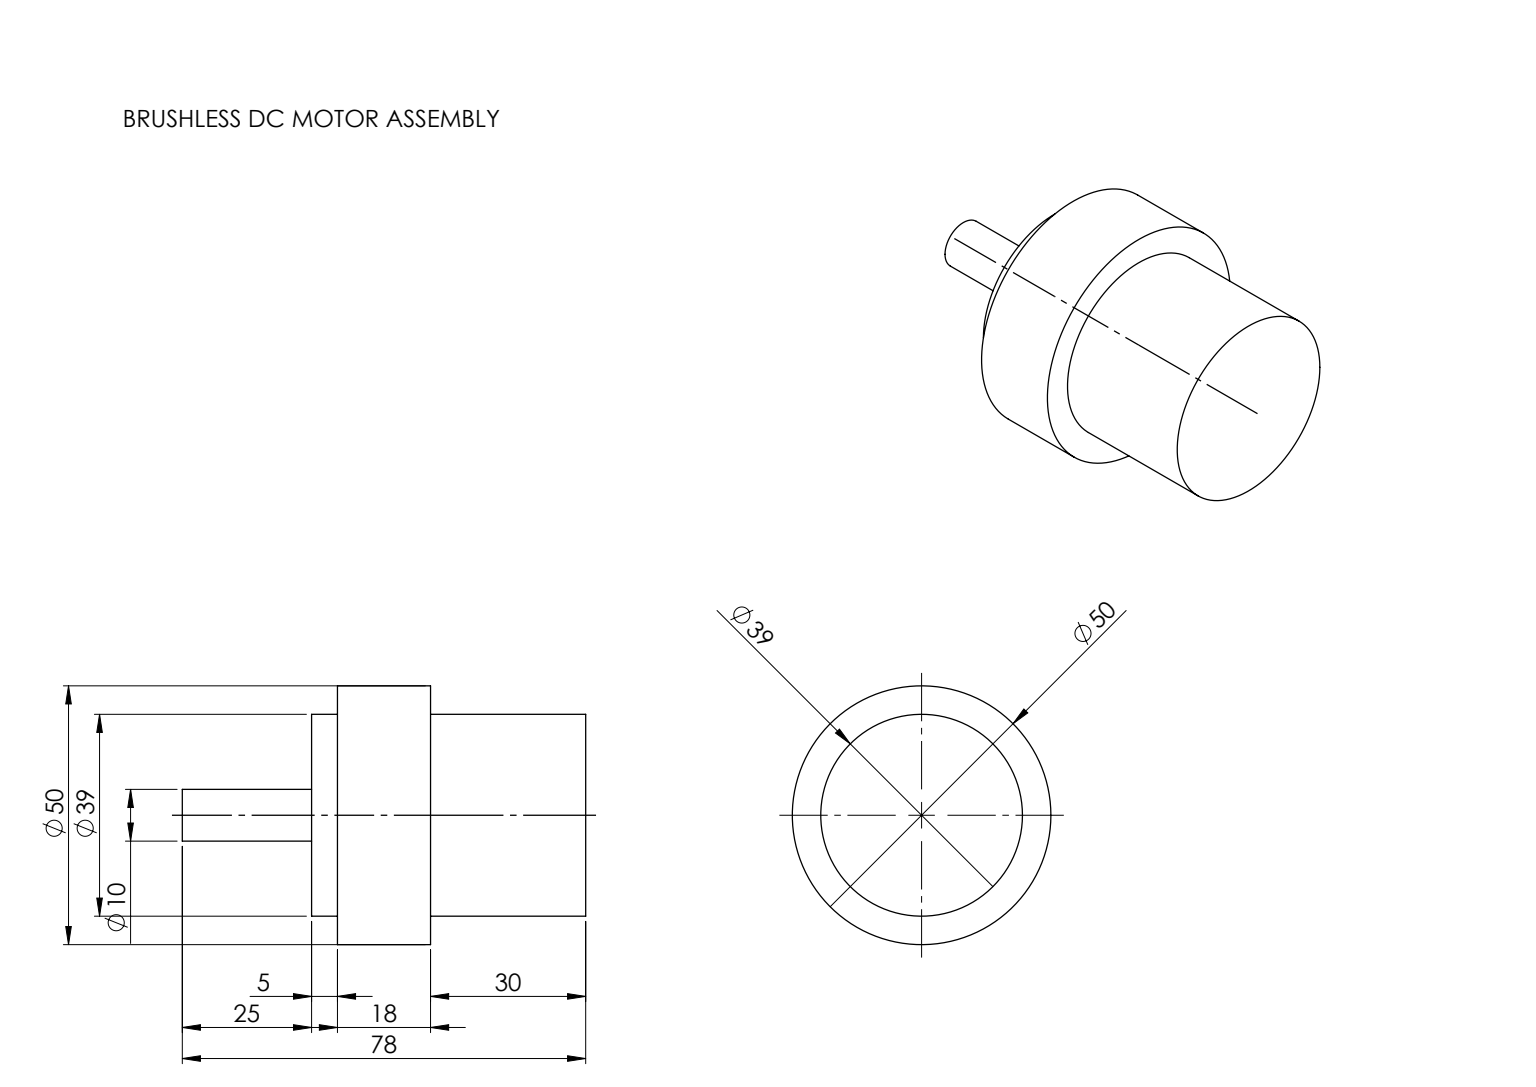
ISO-10303-21;
HEADER;
FILE_DESCRIPTION (('STEP AP214'),
    '1' );
FILE_NAME ('Brushless DC Motor Assembly.step',
    '2026-10-05T20:22:16',
    ( '' ),
    ( '' ),
    'SwSTEP 2.0',
    'SolidWorks 2026',
    '' );
FILE_SCHEMA (( 'AUTOMOTIVE_DESIGN' ));
ENDSEC;

DATA;
#83=ORIENTED_EDGE ( 'NONE', *, *, #15385, .F. ) ;
#148=( LENGTH_UNIT ( ) NAMED_UNIT ( * ) SI_UNIT ( .MILLI., .METRE. ) );
#153=CYLINDRICAL_SURFACE ( 'NONE', #9538, 24.99999999999999645 ) ;
#181=CARTESIAN_POINT ( 'NONE',  ( -50.00000000000000000, 171.6227766016838245, 0.000000000000000000 ) ) ;
#284=CARTESIAN_POINT ( 'NONE',  ( -68.00000000000000000, 171.6227766016838245, 24.99999999999999289 ) ) ;
#327=PRESENTATION_STYLE_ASSIGNMENT (( #16528 ) ) ;
#375=CARTESIAN_POINT ( 'NONE',  ( -68.00000000000000000, 171.6227766016838245, -19.49999999999999645 ) ) ;
#389=EDGE_LOOP ( 'NONE', ( #662, #9822, #5339, #17357 ) ) ;
#493=ORIENTED_EDGE ( 'NONE', *, *, #9337, .F. ) ;
#506=VECTOR ( 'NONE', #763, 1000.000000000000000 ) ;
#507=ORIENTED_EDGE ( 'NONE', *, *, #5137, .F. ) ;
#527=DIRECTION ( 'NONE',  ( 1.000000000000000000, -0.000000000000000000, -0.000000000000000000 ) ) ;
#616=DIRECTION ( 'NONE',  ( 0.000000000000000000, 0.000000000000000000, 1.000000000000000000 ) ) ;
#628=EDGE_CURVE ( 'NONE', #9656, #12025, #15580, .T. ) ;
#636=CARTESIAN_POINT ( 'NONE',  ( -68.00000000000000000, 171.6227766016838245, 0.000000000000000000 ) ) ;
#662=ORIENTED_EDGE ( 'NONE', *, *, #10245, .F. ) ;
#746=DIRECTION ( 'NONE',  ( 0.000000000000000000, 0.000000000000000000, 1.000000000000000000 ) ) ;
#751=DIRECTION ( 'NONE',  ( -1.000000000000000000, 0.000000000000000000, 0.000000000000000000 ) ) ;
#763=DIRECTION ( 'NONE',  ( -1.000000000000000000, -0.000000000000000000, -0.000000000000000000 ) ) ;
#908=ORIENTED_EDGE ( 'NONE', *, *, #8104, .T. ) ;
#928=ORIENTED_EDGE ( 'NONE', *, *, #4621, .F. ) ;
#989=FACE_OUTER_BOUND ( 'NONE', #6924, .T. ) ;
#992=DIRECTION ( 'NONE',  ( -1.000000000000000000, 0.000000000000000000, 0.000000000000000000 ) ) ;
#1039=AXIS2_PLACEMENT_3D ( 'NONE', #16734, #11404, #12560 ) ;
#1159=ADVANCED_FACE ( 'NONE', ( #4225 ), #17507, .T. ) ;
#1236=DIRECTION ( 'NONE',  ( 1.000000000000000000, 0.000000000000000000, -0.000000000000000000 ) ) ;
#1281=DIRECTION ( 'NONE',  ( 0.000000000000000000, 0.000000000000000000, 1.000000000000000000 ) ) ;
#1300=AXIS2_PLACEMENT_3D ( 'NONE', #2966, #10847, #2802 ) ;
#1345=COLOUR_RGB ( '', 0.08235294, 0.09019608, 0.10196078) ;
#1351=PRODUCT_DEFINITION ( 'UNKNOWN', '', #8975, #12448 ) ;
#1374=ORIENTED_EDGE ( 'NONE', *, *, #14927, .T. ) ;
#1493=PLANE ( 'NONE',  #4122 ) ;
#1524=DIRECTION ( 'NONE',  ( 1.000000000000000000, 0.000000000000000000, 0.000000000000000000 ) ) ;
#1543=CARTESIAN_POINT ( 'NONE',  ( -73.00000000000001421, 171.6227766016838245, 5.000000000000006217 ) ) ;
#1546=FACE_OUTER_BOUND ( 'NONE', #389, .T. ) ;
#1562=SURFACE_SIDE_STYLE ('',( #10778 ) ) ;
#1574=EDGE_CURVE ( 'NONE', #14903, #9038, #2433, .T. ) ;
#1722=AXIS2_PLACEMENT_3D ( 'NONE', #2794, #16251, #2704 ) ;
#1774=ORIENTED_EDGE ( 'NONE', *, *, #8939, .F. ) ;
#1789=CARTESIAN_POINT ( 'NONE',  ( -68.00000000000000000, 171.6227766016838245, -25.00000000000000000 ) ) ;
#1833=PLANE ( 'NONE',  #14966 ) ;
#1897=CARTESIAN_POINT ( 'NONE',  ( -50.00000000000000000, 171.6227766016838245, -2.296212748401287183E-15 ) ) ;
#1995=CARTESIAN_POINT ( 'NONE',  ( -20.00000000000000355, 171.6227766016838245, 19.49999999999998934 ) ) ;
#2011=AXIS2_PLACEMENT_3D ( 'NONE', #636, #9923, #3019 ) ;
#2016=CARTESIAN_POINT ( 'NONE',  ( -73.00000000000001421, 171.6227766016838245, 19.49999999999999645 ) ) ;
#2021=ADVANCED_FACE ( 'NONE', ( #14578 ), #2450, .T. ) ;
#2078=ORIENTED_EDGE ( 'NONE', *, *, #17126, .F. ) ;
#2104=ORIENTED_EDGE ( 'NONE', *, *, #6682, .T. ) ;
#2130=CARTESIAN_POINT ( 'NONE',  ( -138.7106781186547266, 171.6227766016838245, -25.00000000000000000 ) ) ;
#2157=DIRECTION ( 'NONE',  ( 0.000000000000000000, 0.000000000000000000, 1.000000000000000000 ) ) ;
#2167=ORIENTED_EDGE ( 'NONE', *, *, #4621, .T. ) ;
#2199=( LENGTH_UNIT ( ) NAMED_UNIT ( * ) SI_UNIT ( .MILLI., .METRE. ) );
#2383=DIRECTION ( 'NONE',  ( 0.000000000000000000, 0.000000000000000000, 1.000000000000000000 ) ) ;
#2387=AXIS2_PLACEMENT_3D ( 'NONE', #8252, #1524, #6920 ) ;
#2393=ORIENTED_EDGE ( 'NONE', *, *, #14927, .F. ) ;
#2433=CIRCLE ( 'NONE', #6680, 19.49999999999999645 ) ;
#2450=CYLINDRICAL_SURFACE ( 'NONE', #12720, 24.99999999999999645 ) ;
#2520=EDGE_CURVE ( 'NONE', #6066, #5020, #9110, .T. ) ;
#2642=EDGE_LOOP ( 'NONE', ( #17068, #9628, #2768, #7721 ) ) ;
#2652=ORIENTED_EDGE ( 'NONE', *, *, #10245, .T. ) ;
#2690=CARTESIAN_POINT ( 'NONE',  ( -50.00000000000000000, 171.6227766016838245, -19.49999999999998934 ) ) ;
#2704=DIRECTION ( 'NONE',  ( 0.000000000000000000, 0.000000000000000000, -1.000000000000000000 ) ) ;
#2707=CIRCLE ( 'NONE', #12597, 19.49999999999998934 ) ;
#2727=CLOSED_SHELL ( 'NONE', ( #6033, #12737, #9025, #2021, #13496, #6623, #3604, #8684, #14834, #3442, #10301, #1159, #11380 ) ) ;
#2768=ORIENTED_EDGE ( 'NONE', *, *, #7492, .T. ) ;
#2790=SHAPE_DEFINITION_REPRESENTATION ( #14917, #17442 ) ;
#2794=CARTESIAN_POINT ( 'NONE',  ( -73.00000000000001421, 171.6227766016838245, 0.000000000000000000 ) ) ;
#2802=DIRECTION ( 'NONE',  ( 0.000000000000000000, 0.000000000000000000, -1.000000000000000000 ) ) ;
#2923=DIRECTION ( 'NONE',  ( 0.000000000000000000, 0.000000000000000000, -1.000000000000000000 ) ) ;
#2936=DIRECTION ( 'NONE',  ( -1.000000000000000000, -0.000000000000000000, -0.000000000000000000 ) ) ;
#2966=CARTESIAN_POINT ( 'NONE',  ( -50.00000000000000000, 171.6227766016838245, -2.296212748401287183E-15 ) ) ;
#2969=DIRECTION ( 'NONE',  ( 0.000000000000000000, 0.000000000000000000, -1.000000000000000000 ) ) ;
#2974=( NAMED_UNIT ( * ) PLANE_ANGLE_UNIT ( ) SI_UNIT ( $, .RADIAN. ) );
#3019=DIRECTION ( 'NONE',  ( 0.000000000000000000, 0.000000000000000000, 1.000000000000000000 ) ) ;
#3082=CIRCLE ( 'NONE', #13271, 24.99999999999999645 ) ;
#3103=ORIENTED_EDGE ( 'NONE', *, *, #7492, .F. ) ;
#3189=EDGE_LOOP ( 'NONE', ( #2167, #14857 ) ) ;
#3217=VERTEX_POINT ( 'NONE', #7731 ) ;
#3225=VERTEX_POINT ( 'NONE', #7568 ) ;
#3227=DIRECTION ( 'NONE',  ( 1.000000000000000000, -0.000000000000000000, -0.000000000000000000 ) ) ;
#3256=COLOUR_RGB ( '', 0.08235294, 0.09019608, 0.10196078) ;
#3280=CARTESIAN_POINT ( 'NONE',  ( -73.00000000000001421, 171.6227766016838245, 0.000000000000000000 ) ) ;
#3308=CIRCLE ( 'NONE', #7822, 5.000000000000006217 ) ;
#3377=CIRCLE ( 'NONE', #6186, 5.000000000000006217 ) ;
#3407=CYLINDRICAL_SURFACE ( 'NONE', #14893, 19.49999999999998934 ) ;
#3431=LINE ( 'NONE', #2016, #6489 ) ;
#3442=ADVANCED_FACE ( 'NONE', ( #9595 ), #14998, .T. ) ;
#3530=VECTOR ( 'NONE', #14519, 1000.000000000000000 ) ;
#3583=AXIS2_PLACEMENT_3D ( 'NONE', #5482, #6893, #8222 ) ;
#3604=ADVANCED_FACE ( 'NONE', ( #11764, #13191 ), #4001, .F. ) ;
#3626=AXIS2_PLACEMENT_3D ( 'NONE', #13286, #1236, #2383 ) ;
#3652=ORIENTED_EDGE ( 'NONE', *, *, #5137, .T. ) ;
#3715=CIRCLE ( 'NONE', #4287, 5.000000000000006217 ) ;
#3819=DIRECTION ( 'NONE',  ( 0.000000000000000000, 0.000000000000000000, -1.000000000000000000 ) ) ;
#3834=CYLINDRICAL_SURFACE ( 'NONE', #12341, 5.000000000000006217 ) ;
#3877=EDGE_LOOP ( 'NONE', ( #4904, #2393 ) ) ;
#3989=AXIS2_PLACEMENT_3D ( 'NONE', #5717, #3227, #11105 ) ;
#4001=PLANE ( 'NONE',  #3626 ) ;
#4025=DIRECTION ( 'NONE',  ( 0.000000000000000000, 0.000000000000000000, -1.000000000000000000 ) ) ;
#4122=AXIS2_PLACEMENT_3D ( 'NONE', #9711, #9626, #4240 ) ;
#4137=FILL_AREA_STYLE_COLOUR ( '', #1345 ) ;
#4154=ORIENTED_EDGE ( 'NONE', *, *, #8876, .T. ) ;
#4159=AXIS2_PLACEMENT_3D ( 'NONE', #11837, #11661, #10329 ) ;
#4173=CIRCLE ( 'NONE', #4159, 5.000000000000006217 ) ;
#4175=DIRECTION ( 'NONE',  ( 1.000000000000000000, 0.000000000000000000, 0.000000000000000000 ) ) ;
#4225=FACE_OUTER_BOUND ( 'NONE', #9263, .T. ) ;
#4240=DIRECTION ( 'NONE',  ( 0.000000000000000000, 0.000000000000000000, 1.000000000000000000 ) ) ;
#4243=ORIENTED_EDGE ( 'NONE', *, *, #17126, .T. ) ;
#4287=AXIS2_PLACEMENT_3D ( 'NONE', #15608, #992, #9133 ) ;
#4401=( NAMED_UNIT ( * ) SI_UNIT ( $, .STERADIAN. ) SOLID_ANGLE_UNIT ( ) );
#4507=ORIENTED_EDGE ( 'NONE', *, *, #7212, .F. ) ;
#4571=PLANE ( 'NONE',  #10997 ) ;
#4621=EDGE_CURVE ( 'NONE', #5464, #5020, #3082, .T. ) ;
#4692=( NAMED_UNIT ( * ) SI_UNIT ( $, .STERADIAN. ) SOLID_ANGLE_UNIT ( ) );
#4720=VERTEX_POINT ( 'NONE', #6227 ) ;
#4750=ORIENTED_EDGE ( 'NONE', *, *, #1574, .F. ) ;
#4904=ORIENTED_EDGE ( 'NONE', *, *, #13206, .F. ) ;
#4938=DIRECTION ( 'NONE',  ( 1.000000000000000000, 0.000000000000000000, 0.000000000000000000 ) ) ;
#4992=VECTOR ( 'NONE', #8844, 1000.000000000000000 ) ;
#5020=VERTEX_POINT ( 'NONE', #12936 ) ;
#5032=SURFACE_STYLE_USAGE ( .BOTH. , #15836 ) ;
#5137=EDGE_CURVE ( 'NONE', #6998, #13633, #15759, .T. ) ;
#5139=DIRECTION ( 'NONE',  ( 1.000000000000000000, 0.000000000000000000, 0.000000000000000000 ) ) ;
#5231=DIRECTION ( 'NONE',  ( 0.000000000000000000, 0.000000000000000000, 1.000000000000000000 ) ) ;
#5271=EDGE_CURVE ( 'NONE', #3217, #5676, #17416, .T. ) ;
#5339=ORIENTED_EDGE ( 'NONE', *, *, #8939, .T. ) ;
#5378=CARTESIAN_POINT ( 'NONE',  ( -98.00000000000000000, 171.6227766016838245, 0.000000000000000000 ) ) ;
#5396=DIRECTION ( 'NONE',  ( 0.000000000000000000, 0.000000000000000000, -1.000000000000000000 ) ) ;
#5420=CARTESIAN_POINT ( 'NONE',  ( -20.00000000000000355, 171.6227766016838245, 0.000000000000000000 ) ) ;
#5464=VERTEX_POINT ( 'NONE', #15892 ) ;
#5482=CARTESIAN_POINT ( 'NONE',  ( 0.000000000000000000, 0.000000000000000000, 0.000000000000000000 ) ) ;
#5593=PRODUCT ( 'Brushless DC Motor Assembly', 'Brushless DC Motor Assembly', '', ( #12343 ) ) ;
#5676=VERTEX_POINT ( 'NONE', #1543 ) ;
#5717=CARTESIAN_POINT ( 'NONE',  ( -73.00000000000001421, 171.6227766016838245, 0.000000000000000000 ) ) ;
#6008=EDGE_LOOP ( 'NONE', ( #7802, #11194, #4243, #8727 ) ) ;
#6033=ADVANCED_FACE ( 'NONE', ( #989 ), #3834, .T. ) ;
#6066=VERTEX_POINT ( 'NONE', #284 ) ;
#6160=ORIENTED_EDGE ( 'NONE', *, *, #10501, .F. ) ;
#6185=CARTESIAN_POINT ( 'NONE',  ( -20.00000000000000355, 171.6227766016838245, 0.000000000000000000 ) ) ;
#6186=AXIS2_PLACEMENT_3D ( 'NONE', #15789, #9059, #2157 ) ;
#6227=CARTESIAN_POINT ( 'NONE',  ( -68.00000000000000000, 171.6227766016838245, 19.49999999999999645 ) ) ;
#6489=VECTOR ( 'NONE', #11648, 1000.000000000000000 ) ;
#6623=ADVANCED_FACE ( 'NONE', ( #13817, #13907 ), #7163, .T. ) ;
#6657=EDGE_CURVE ( 'NONE', #3217, #6998, #3308, .T. ) ;
#6680=AXIS2_PLACEMENT_3D ( 'NONE', #3280, #8686, #14092 ) ;
#6682=EDGE_CURVE ( 'NONE', #14903, #15136, #9816, .T. ) ;
#6770=ORIENTED_EDGE ( 'NONE', *, *, #9337, .T. ) ;
#6837=ORIENTED_EDGE ( 'NONE', *, *, #15532, .F. ) ;
#6884=DIRECTION ( 'NONE',  ( -1.000000000000000000, -0.000000000000000000, -0.000000000000000000 ) ) ;
#6893=DIRECTION ( 'NONE',  ( 0.000000000000000000, 0.000000000000000000, 1.000000000000000000 ) ) ;
#6920=DIRECTION ( 'NONE',  ( 0.000000000000000000, 0.000000000000000000, -1.000000000000000000 ) ) ;
#6924=EDGE_LOOP ( 'NONE', ( #7855, #8965, #1374, #507 ) ) ;
#6997=FILL_AREA_STYLE ('',( #16395 ) ) ;
#6998=VERTEX_POINT ( 'NONE', #14125 ) ;
#7163=PLANE ( 'NONE',  #1039 ) ;
#7212=EDGE_CURVE ( 'NONE', #6066, #10900, #11140, .T. ) ;
#7281=EDGE_CURVE ( 'NONE', #3225, #12025, #12010, .T. ) ;
#7352=AXIS2_PLACEMENT_3D ( 'NONE', #9535, #6884, #5396 ) ;
#7492=EDGE_CURVE ( 'NONE', #10900, #5464, #14263, .T. ) ;
#7568=CARTESIAN_POINT ( 'NONE',  ( -50.00000000000000000, 171.6227766016838245, 19.49999999999998934 ) ) ;
#7721=ORIENTED_EDGE ( 'NONE', *, *, #11731, .F. ) ;
#7731=CARTESIAN_POINT ( 'NONE',  ( -98.00000000000000000, 171.6227766016838245, 5.000000000000006217 ) ) ;
#7802=ORIENTED_EDGE ( 'NONE', *, *, #628, .F. ) ;
#7822=AXIS2_PLACEMENT_3D ( 'NONE', #9981, #11231, #616 ) ;
#7846=DIRECTION ( 'NONE',  ( 1.000000000000000000, 0.000000000000000000, 0.000000000000000000 ) ) ;
#7855=ORIENTED_EDGE ( 'NONE', *, *, #6657, .F. ) ;
#8002=CARTESIAN_POINT ( 'NONE',  ( -20.00000000000000355, 171.6227766016838245, 0.000000000000000000 ) ) ;
#8046=CARTESIAN_POINT ( 'NONE',  ( -138.7106781186547266, 171.6227766016838245, 24.99999999999999289 ) ) ;
#8104=EDGE_CURVE ( 'NONE', #10900, #6066, #14978, .T. ) ;
#8115=MECHANICAL_DESIGN_GEOMETRIC_PRESENTATION_REPRESENTATION('',(#9239),#16325);
#8118=ORIENTED_EDGE ( 'NONE', *, *, #15385, .T. ) ;
#8222=DIRECTION ( 'NONE',  ( 1.000000000000000000, 0.000000000000000000, 0.000000000000000000 ) ) ;
#8252=CARTESIAN_POINT ( 'NONE',  ( -50.00000000000000000, 171.6227766016838245, 0.000000000000000000 ) ) ;
#8262=EDGE_LOOP ( 'NONE', ( #6770, #13870 ) ) ;
#8284=( NAMED_UNIT ( * ) SI_UNIT ( $, .STERADIAN. ) SOLID_ANGLE_UNIT ( ) );
#8291=CARTESIAN_POINT ( 'NONE',  ( -138.7106781186547266, 171.6227766016838245, -2.296212748401287183E-15 ) ) ;
#8321=AXIS2_PLACEMENT_3D ( 'NONE', #11079, #2936, #4025 ) ;
#8373=( LENGTH_UNIT ( ) NAMED_UNIT ( * ) SI_UNIT ( .MILLI., .METRE. ) );
#8456=FACE_OUTER_BOUND ( 'NONE', #11793, .T. ) ;
#8479=DIRECTION ( 'NONE',  ( 0.000000000000000000, 0.000000000000000000, -1.000000000000000000 ) ) ;
#8517=CARTESIAN_POINT ( 'NONE',  ( -20.00000000000000355, 171.6227766016838245, -19.49999999999998934 ) ) ;
#8543=CARTESIAN_POINT ( 'NONE',  ( -73.00000000000001421, 171.6227766016838245, 0.000000000000000000 ) ) ;
#8684=ADVANCED_FACE ( 'NONE', ( #8456 ), #15084, .T. ) ;
#8686=DIRECTION ( 'NONE',  ( -1.000000000000000000, 0.000000000000000000, 0.000000000000000000 ) ) ;
#8727=ORIENTED_EDGE ( 'NONE', *, *, #7281, .T. ) ;
#8775=UNCERTAINTY_MEASURE_WITH_UNIT (LENGTH_MEASURE( 1.000000000000000082E-05 ), #148, 'distance_accuracy_value', 'NONE');
#8844=DIRECTION ( 'NONE',  ( -1.000000000000000000, -0.000000000000000000, -0.000000000000000000 ) ) ;
#8876=EDGE_CURVE ( 'NONE', #15136, #4720, #10204, .T. ) ;
#8918=CIRCLE ( 'NONE', #1300, 24.99999999999999645 ) ;
#8939=EDGE_CURVE ( 'NONE', #4720, #15136, #16998, .T. ) ;
#8965=ORIENTED_EDGE ( 'NONE', *, *, #5271, .T. ) ;
#8975=PRODUCT_DEFINITION_FORMATION_WITH_SPECIFIED_SOURCE ( 'ANY', '', #5593, .NOT_KNOWN. ) ;
#9025=ADVANCED_FACE ( 'NONE', ( #1546 ), #10761, .T. ) ;
#9038=VERTEX_POINT ( 'NONE', #13413 ) ;
#9059=DIRECTION ( 'NONE',  ( -1.000000000000000000, 0.000000000000000000, 0.000000000000000000 ) ) ;
#9110=LINE ( 'NONE', #8046, #13864 ) ;
#9133=DIRECTION ( 'NONE',  ( 0.000000000000000000, 0.000000000000000000, 1.000000000000000000 ) ) ;
#9147=UNCERTAINTY_MEASURE_WITH_UNIT (LENGTH_MEASURE( 1.000000000000000082E-05 ), #2199, 'distance_accuracy_value', 'NONE');
#9212=DIRECTION ( 'NONE',  ( 1.000000000000000000, 0.000000000000000000, 0.000000000000000000 ) ) ;
#9239=STYLED_ITEM ( 'NONE', ( #327 ), #16081 ) ;
#9263=EDGE_LOOP ( 'NONE', ( #13654, #493, #3652, #17284 ) ) ;
#9337=EDGE_CURVE ( 'NONE', #6998, #3217, #3715, .T. ) ;
#9349=AXIS2_PLACEMENT_3D ( 'NONE', #8002, #12083, #1281 ) ;
#9535=CARTESIAN_POINT ( 'NONE',  ( -68.00000000000000000, 171.6227766016838245, -2.296212748401287183E-15 ) ) ;
#9538=AXIS2_PLACEMENT_3D ( 'NONE', #8291, #13699, #12546 ) ;
#9595=FACE_OUTER_BOUND ( 'NONE', #6008, .T. ) ;
#9611=DIRECTION ( 'NONE',  ( 1.000000000000000000, -0.000000000000000000, -0.000000000000000000 ) ) ;
#9612=ORIENTED_EDGE ( 'NONE', *, *, #2520, .T. ) ;
#9615=FILL_AREA_STYLE ('',( #4137 ) ) ;
#9626=DIRECTION ( 'NONE',  ( -1.000000000000000000, 0.000000000000000000, 0.000000000000000000 ) ) ;
#9628=ORIENTED_EDGE ( 'NONE', *, *, #8104, .F. ) ;
#9656=VERTEX_POINT ( 'NONE', #8517 ) ;
#9711=CARTESIAN_POINT ( 'NONE',  ( -98.00000000000000000, 171.6227766016838245, 0.000000000000000000 ) ) ;
#9791=SHAPE_REPRESENTATION_RELATIONSHIP ( 'NONE' , 'NONE' ,  #17442, #16081 ) ;
#9803=FACE_OUTER_BOUND ( 'NONE', #8262, .T. ) ;
#9816=LINE ( 'NONE', #11326, #15952 ) ;
#9822=ORIENTED_EDGE ( 'NONE', *, *, #10501, .T. ) ;
#9869=DIRECTION ( 'NONE',  ( -1.000000000000000000, 0.000000000000000000, 0.000000000000000000 ) ) ;
#9923=DIRECTION ( 'NONE',  ( -1.000000000000000000, 0.000000000000000000, 0.000000000000000000 ) ) ;
#9954=DIRECTION ( 'NONE',  ( 0.000000000000000000, 0.000000000000000000, 1.000000000000000000 ) ) ;
#9981=CARTESIAN_POINT ( 'NONE',  ( -98.00000000000000000, 171.6227766016838245, 0.000000000000000000 ) ) ;
#9984=DIRECTION ( 'NONE',  ( 0.000000000000000000, 0.000000000000000000, -1.000000000000000000 ) ) ;
#10016=EDGE_CURVE ( 'NONE', #13808, #9656, #16935, .T. ) ;
#10154=CIRCLE ( 'NONE', #17230, 19.49999999999998934 ) ;
#10185=UNCERTAINTY_MEASURE_WITH_UNIT (LENGTH_MEASURE( 1.000000000000000082E-05 ), #8373, 'distance_accuracy_value', 'NONE');
#10204=CIRCLE ( 'NONE', #10765, 19.49999999999999645 ) ;
#10245=EDGE_CURVE ( 'NONE', #9038, #14903, #13281, .T. ) ;
#10253=( NAMED_UNIT ( * ) PLANE_ANGLE_UNIT ( ) SI_UNIT ( $, .RADIAN. ) );
#10301=ADVANCED_FACE ( 'NONE', ( #15295 ), #1833, .T. ) ;
#10329=DIRECTION ( 'NONE',  ( 0.000000000000000000, 0.000000000000000000, 1.000000000000000000 ) ) ;
#10333=SURFACE_STYLE_FILL_AREA ( #6997 ) ;
#10449=DIRECTION ( 'NONE',  ( 1.000000000000000000, 0.000000000000000000, 0.000000000000000000 ) ) ;
#10501=EDGE_CURVE ( 'NONE', #9038, #4720, #3431, .T. ) ;
#10596=CARTESIAN_POINT ( 'NONE',  ( -73.00000000000001421, 171.6227766016838245, 0.000000000000000000 ) ) ;
#10643=CARTESIAN_POINT ( 'NONE',  ( -98.00000000000000000, 171.6227766016838245, 0.000000000000000000 ) ) ;
#10652=EDGE_LOOP ( 'NONE', ( #13129, #2652 ) ) ;
#10761=CYLINDRICAL_SURFACE ( 'NONE', #1722, 19.49999999999999645 ) ;
#10765=AXIS2_PLACEMENT_3D ( 'NONE', #17359, #751, #5231 ) ;
#10778=SURFACE_STYLE_FILL_AREA ( #9615 ) ;
#10783=EDGE_LOOP ( 'NONE', ( #13984, #6837 ) ) ;
#10847=DIRECTION ( 'NONE',  ( 1.000000000000000000, 0.000000000000000000, 0.000000000000000000 ) ) ;
#10880=MECHANICAL_DESIGN_GEOMETRIC_PRESENTATION_REPRESENTATION('',(#11453),#16269);
#10900=VERTEX_POINT ( 'NONE', #1789 ) ;
#10997=AXIS2_PLACEMENT_3D ( 'NONE', #8543, #9869, #9954 ) ;
#11079=CARTESIAN_POINT ( 'NONE',  ( -68.00000000000000000, 171.6227766016838245, -2.296212748401287183E-15 ) ) ;
#11105=DIRECTION ( 'NONE',  ( 0.000000000000000000, 0.000000000000000000, -1.000000000000000000 ) ) ;
#11108=FACE_OUTER_BOUND ( 'NONE', #10652, .T. ) ;
#11140=CIRCLE ( 'NONE', #8321, 24.99999999999999645 ) ;
#11181=MANIFOLD_SOLID_BREP ( 'Boss-Extrude4', #2727 ) ;
#11194=ORIENTED_EDGE ( 'NONE', *, *, #10016, .F. ) ;
#11231=DIRECTION ( 'NONE',  ( -1.000000000000000000, 0.000000000000000000, 0.000000000000000000 ) ) ;
#11276=DIRECTION ( 'NONE',  ( 0.000000000000000000, 0.000000000000000000, -1.000000000000000000 ) ) ;
#11326=CARTESIAN_POINT ( 'NONE',  ( -73.00000000000001421, 171.6227766016838245, -19.49999999999999645 ) ) ;
#11380=ADVANCED_FACE ( 'NONE', ( #9803 ), #1493, .T. ) ;
#11400=EDGE_LOOP ( 'NONE', ( #908, #15368 ) ) ;
#11404=DIRECTION ( 'NONE',  ( 1.000000000000000000, 0.000000000000000000, 0.000000000000000000 ) ) ;
#11453=STYLED_ITEM ( 'NONE', ( #14331 ), #11181 ) ;
#11648=DIRECTION ( 'NONE',  ( 1.000000000000000000, -0.000000000000000000, -0.000000000000000000 ) ) ;
#11655=CARTESIAN_POINT ( 'NONE',  ( -138.7106781186547266, 171.6227766016838245, -2.296212748401287183E-15 ) ) ;
#11661=DIRECTION ( 'NONE',  ( -1.000000000000000000, 0.000000000000000000, 0.000000000000000000 ) ) ;
#11731=EDGE_CURVE ( 'NONE', #5020, #5464, #8918, .T. ) ;
#11764=FACE_BOUND ( 'NONE', #14054, .T. ) ;
#11793=EDGE_LOOP ( 'NONE', ( #6160, #4750, #2104, #4154 ) ) ;
#11837=CARTESIAN_POINT ( 'NONE',  ( -73.00000000000001421, 171.6227766016838245, 0.000000000000000000 ) ) ;
#11840=APPLICATION_CONTEXT ( 'automotive_design' ) ;
#12010=CIRCLE ( 'NONE', #2387, 19.49999999999998934 ) ;
#12025=VERTEX_POINT ( 'NONE', #2690 ) ;
#12078=( GEOMETRIC_REPRESENTATION_CONTEXT ( 3 ) GLOBAL_UNCERTAINTY_ASSIGNED_CONTEXT ( ( #8775 ) ) GLOBAL_UNIT_ASSIGNED_CONTEXT ( ( #148, #2974, #8284 ) ) REPRESENTATION_CONTEXT ( 'NONE', 'WORKASPACE' ) );
#12083=DIRECTION ( 'NONE',  ( -1.000000000000000000, -0.000000000000000000, -0.000000000000000000 ) ) ;
#12111=CARTESIAN_POINT ( 'NONE',  ( -98.00000000000000000, 171.6227766016838245, 5.000000000000006217 ) ) ;
#12116=FACE_OUTER_BOUND ( 'NONE', #2642, .T. ) ;
#12205=DIRECTION ( 'NONE',  ( 1.000000000000000000, 0.000000000000000000, 0.000000000000000000 ) ) ;
#12341=AXIS2_PLACEMENT_3D ( 'NONE', #10643, #16318, #17469 ) ;
#12343=PRODUCT_CONTEXT ( 'NONE', #11840, 'mechanical' ) ;
#12448=PRODUCT_DEFINITION_CONTEXT ( 'detailed design', #12523, 'design' ) ;
#12523=APPLICATION_CONTEXT ( 'automotive_design' ) ;
#12546=DIRECTION ( 'NONE',  ( 0.000000000000000000, 0.000000000000000000, -1.000000000000000000 ) ) ;
#12547=CARTESIAN_POINT ( 'NONE',  ( -20.00000000000000355, 171.6227766016838245, 0.000000000000000000 ) ) ;
#12560=DIRECTION ( 'NONE',  ( 0.000000000000000000, 0.000000000000000000, -1.000000000000000000 ) ) ;
#12597=AXIS2_PLACEMENT_3D ( 'NONE', #181, #9212, #2923 ) ;
#12709=FACE_BOUND ( 'NONE', #3877, .T. ) ;
#12720=AXIS2_PLACEMENT_3D ( 'NONE', #11655, #7846, #17057 ) ;
#12737=ADVANCED_FACE ( 'NONE', ( #15526 ), #3407, .T. ) ;
#12936=CARTESIAN_POINT ( 'NONE',  ( -50.00000000000000000, 171.6227766016838245, 24.99999999999999289 ) ) ;
#13129=ORIENTED_EDGE ( 'NONE', *, *, #1574, .T. ) ;
#13191=FACE_OUTER_BOUND ( 'NONE', #11400, .T. ) ;
#13194=CARTESIAN_POINT ( 'NONE',  ( -98.00000000000000000, 171.6227766016838245, -5.000000000000006217 ) ) ;
#13206=EDGE_CURVE ( 'NONE', #13633, #5676, #4173, .T. ) ;
#13246=CARTESIAN_POINT ( 'NONE',  ( -73.00000000000001421, 171.6227766016838245, -5.000000000000006217 ) ) ;
#13267=AXIS2_PLACEMENT_3D ( 'NONE', #6185, #4938, #9984 ) ;
#13271=AXIS2_PLACEMENT_3D ( 'NONE', #1897, #16692, #11276 ) ;
#13281=CIRCLE ( 'NONE', #15817, 19.49999999999999645 ) ;
#13286=CARTESIAN_POINT ( 'NONE',  ( -68.00000000000000000, 171.6227766016838245, 0.000000000000000000 ) ) ;
#13357=DIRECTION ( 'NONE',  ( -1.000000000000000000, 0.000000000000000000, 0.000000000000000000 ) ) ;
#13413=CARTESIAN_POINT ( 'NONE',  ( -73.00000000000001421, 171.6227766016838245, 19.49999999999999645 ) ) ;
#13496=ADVANCED_FACE ( 'NONE', ( #12116 ), #153, .T. ) ;
#13633=VERTEX_POINT ( 'NONE', #13246 ) ;
#13654=ORIENTED_EDGE ( 'NONE', *, *, #5271, .F. ) ;
#13699=DIRECTION ( 'NONE',  ( 1.000000000000000000, 0.000000000000000000, 0.000000000000000000 ) ) ;
#13792=( NAMED_UNIT ( * ) PLANE_ANGLE_UNIT ( ) SI_UNIT ( $, .RADIAN. ) );
#13808=VERTEX_POINT ( 'NONE', #1995 ) ;
#13817=FACE_BOUND ( 'NONE', #10783, .T. ) ;
#13864=VECTOR ( 'NONE', #5139, 1000.000000000000000 ) ;
#13870=ORIENTED_EDGE ( 'NONE', *, *, #6657, .T. ) ;
#13907=FACE_OUTER_BOUND ( 'NONE', #3189, .T. ) ;
#13941=EDGE_LOOP ( 'NONE', ( #16441, #8118 ) ) ;
#13984=ORIENTED_EDGE ( 'NONE', *, *, #7281, .F. ) ;
#14054=EDGE_LOOP ( 'NONE', ( #14527, #1774 ) ) ;
#14092=DIRECTION ( 'NONE',  ( 0.000000000000000000, 0.000000000000000000, 1.000000000000000000 ) ) ;
#14125=CARTESIAN_POINT ( 'NONE',  ( -98.00000000000000000, 171.6227766016838245, -5.000000000000006217 ) ) ;
#14219=CARTESIAN_POINT ( 'NONE',  ( -20.00000000000000355, 171.6227766016838245, 19.49999999999998934 ) ) ;
#14263=LINE ( 'NONE', #2130, #14272 ) ;
#14272=VECTOR ( 'NONE', #10449, 1000.000000000000000 ) ;
#14331=PRESENTATION_STYLE_ASSIGNMENT (( #5032 ) ) ;
#14519=DIRECTION ( 'NONE',  ( 1.000000000000000000, -0.000000000000000000, -0.000000000000000000 ) ) ;
#14527=ORIENTED_EDGE ( 'NONE', *, *, #8876, .F. ) ;
#14578=FACE_OUTER_BOUND ( 'NONE', #17021, .T. ) ;
#14793=EDGE_LOOP ( 'NONE', ( #83, #15360, #14986, #2078 ) ) ;
#14834=ADVANCED_FACE ( 'NONE', ( #12709, #11108 ), #4571, .T. ) ;
#14853=VECTOR ( 'NONE', #17515, 1000.000000000000000 ) ;
#14857=ORIENTED_EDGE ( 'NONE', *, *, #11731, .T. ) ;
#14893=AXIS2_PLACEMENT_3D ( 'NONE', #16860, #17447, #746 ) ;
#14903=VERTEX_POINT ( 'NONE', #15535 ) ;
#14917=PRODUCT_DEFINITION_SHAPE ( 'NONE', 'NONE',  #1351 ) ;
#14927=EDGE_CURVE ( 'NONE', #5676, #13633, #3377, .T. ) ;
#14966=AXIS2_PLACEMENT_3D ( 'NONE', #12547, #12205, #8479 ) ;
#14978=CIRCLE ( 'NONE', #7352, 24.99999999999999645 ) ;
#14986=ORIENTED_EDGE ( 'NONE', *, *, #15532, .T. ) ;
#14998=CYLINDRICAL_SURFACE ( 'NONE', #9349, 19.49999999999998934 ) ;
#15084=CYLINDRICAL_SURFACE ( 'NONE', #3989, 19.49999999999999645 ) ;
#15136=VERTEX_POINT ( 'NONE', #375 ) ;
#15295=FACE_OUTER_BOUND ( 'NONE', #13941, .T. ) ;
#15360=ORIENTED_EDGE ( 'NONE', *, *, #628, .T. ) ;
#15368=ORIENTED_EDGE ( 'NONE', *, *, #7212, .T. ) ;
#15385=EDGE_CURVE ( 'NONE', #9656, #13808, #10154, .T. ) ;
#15399=CARTESIAN_POINT ( 'NONE',  ( -20.00000000000000355, 171.6227766016838245, -19.49999999999998934 ) ) ;
#15455=LINE ( 'NONE', #14219, #506 ) ;
#15526=FACE_OUTER_BOUND ( 'NONE', #14793, .T. ) ;
#15532=EDGE_CURVE ( 'NONE', #12025, #3225, #2707, .T. ) ;
#15535=CARTESIAN_POINT ( 'NONE',  ( -73.00000000000001421, 171.6227766016838245, -19.49999999999999645 ) ) ;
#15555=AXIS2_PLACEMENT_3D ( 'NONE', #5378, #9611, #2969 ) ;
#15580=LINE ( 'NONE', #15399, #4992 ) ;
#15608=CARTESIAN_POINT ( 'NONE',  ( -98.00000000000000000, 171.6227766016838245, 0.000000000000000000 ) ) ;
#15759=LINE ( 'NONE', #13194, #3530 ) ;
#15789=CARTESIAN_POINT ( 'NONE',  ( -73.00000000000001421, 171.6227766016838245, 0.000000000000000000 ) ) ;
#15817=AXIS2_PLACEMENT_3D ( 'NONE', #10596, #13357, #16006 ) ;
#15836=SURFACE_SIDE_STYLE ('',( #10333 ) ) ;
#15892=CARTESIAN_POINT ( 'NONE',  ( -50.00000000000000000, 171.6227766016838245, -25.00000000000000000 ) ) ;
#15952=VECTOR ( 'NONE', #527, 1000.000000000000000 ) ;
#16006=DIRECTION ( 'NONE',  ( 0.000000000000000000, 0.000000000000000000, 1.000000000000000000 ) ) ;
#16081=ADVANCED_BREP_SHAPE_REPRESENTATION ( '', ( #11181, #3583 ), #12078 ) ;
#16251=DIRECTION ( 'NONE',  ( 1.000000000000000000, -0.000000000000000000, -0.000000000000000000 ) ) ;
#16269=( GEOMETRIC_REPRESENTATION_CONTEXT ( 3 ) GLOBAL_UNCERTAINTY_ASSIGNED_CONTEXT ( ( #9147 ) ) GLOBAL_UNIT_ASSIGNED_CONTEXT ( ( #2199, #10253, #4692 ) ) REPRESENTATION_CONTEXT ( 'NONE', 'WORKASPACE' ) );
#16318=DIRECTION ( 'NONE',  ( 1.000000000000000000, -0.000000000000000000, -0.000000000000000000 ) ) ;
#16325=( GEOMETRIC_REPRESENTATION_CONTEXT ( 3 ) GLOBAL_UNCERTAINTY_ASSIGNED_CONTEXT ( ( #10185 ) ) GLOBAL_UNIT_ASSIGNED_CONTEXT ( ( #8373, #13792, #4401 ) ) REPRESENTATION_CONTEXT ( 'NONE', 'WORKASPACE' ) );
#16395=FILL_AREA_STYLE_COLOUR ( '', #3256 ) ;
#16441=ORIENTED_EDGE ( 'NONE', *, *, #10016, .T. ) ;
#16528=SURFACE_STYLE_USAGE ( .BOTH. , #1562 ) ;
#16692=DIRECTION ( 'NONE',  ( 1.000000000000000000, 0.000000000000000000, 0.000000000000000000 ) ) ;
#16734=CARTESIAN_POINT ( 'NONE',  ( -50.00000000000000000, 171.6227766016838245, -2.296212748401287183E-15 ) ) ;
#16860=CARTESIAN_POINT ( 'NONE',  ( -20.00000000000000355, 171.6227766016838245, 0.000000000000000000 ) ) ;
#16935=CIRCLE ( 'NONE', #13267, 19.49999999999998934 ) ;
#16998=CIRCLE ( 'NONE', #2011, 19.49999999999999645 ) ;
#17021=EDGE_LOOP ( 'NONE', ( #4507, #9612, #928, #3103 ) ) ;
#17057=DIRECTION ( 'NONE',  ( 0.000000000000000000, 0.000000000000000000, -1.000000000000000000 ) ) ;
#17068=ORIENTED_EDGE ( 'NONE', *, *, #2520, .F. ) ;
#17126=EDGE_CURVE ( 'NONE', #13808, #3225, #15455, .T. ) ;
#17230=AXIS2_PLACEMENT_3D ( 'NONE', #5420, #4175, #3819 ) ;
#17284=ORIENTED_EDGE ( 'NONE', *, *, #13206, .T. ) ;
#17357=ORIENTED_EDGE ( 'NONE', *, *, #6682, .F. ) ;
#17359=CARTESIAN_POINT ( 'NONE',  ( -68.00000000000000000, 171.6227766016838245, 0.000000000000000000 ) ) ;
#17416=LINE ( 'NONE', #12111, #14853 ) ;
#17442=SHAPE_REPRESENTATION ( 'Brushless DC Motor Assembly', ( #3583 ), #12078 ) ;
#17447=DIRECTION ( 'NONE',  ( -1.000000000000000000, -0.000000000000000000, -0.000000000000000000 ) ) ;
#17469=DIRECTION ( 'NONE',  ( 0.000000000000000000, 0.000000000000000000, -1.000000000000000000 ) ) ;
#17507=CYLINDRICAL_SURFACE ( 'NONE', #15555, 5.000000000000006217 ) ;
#17515=DIRECTION ( 'NONE',  ( 1.000000000000000000, -0.000000000000000000, -0.000000000000000000 ) ) ;
ENDSEC;
END-ISO-10303-21;
